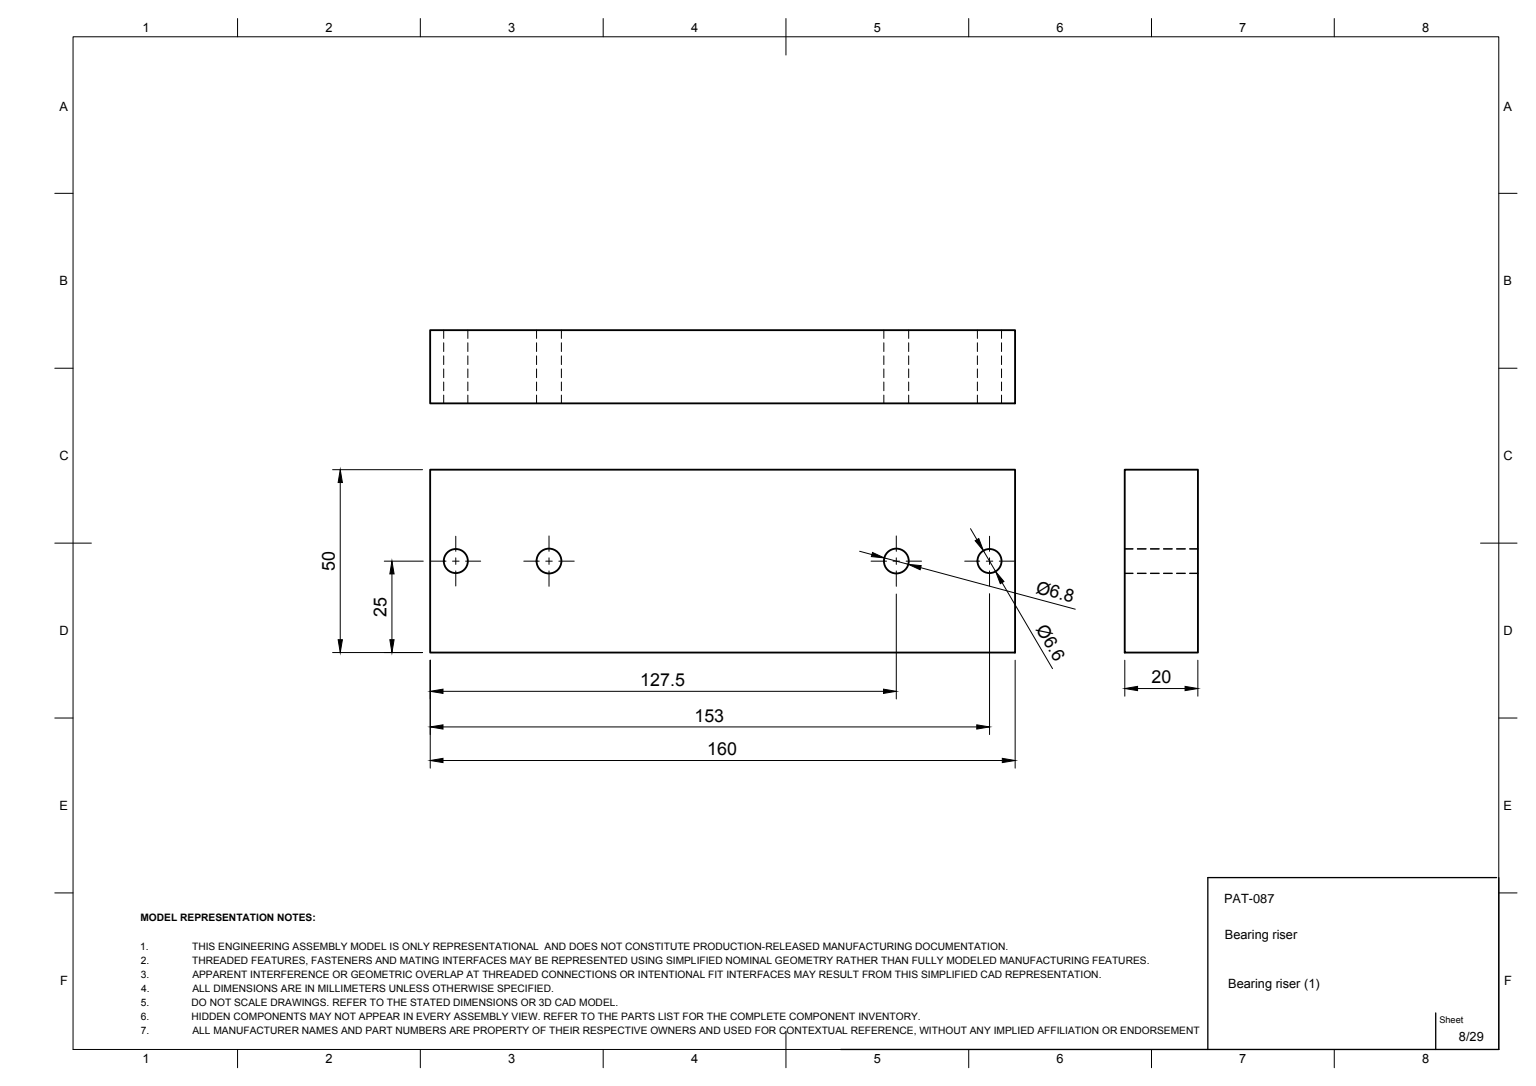
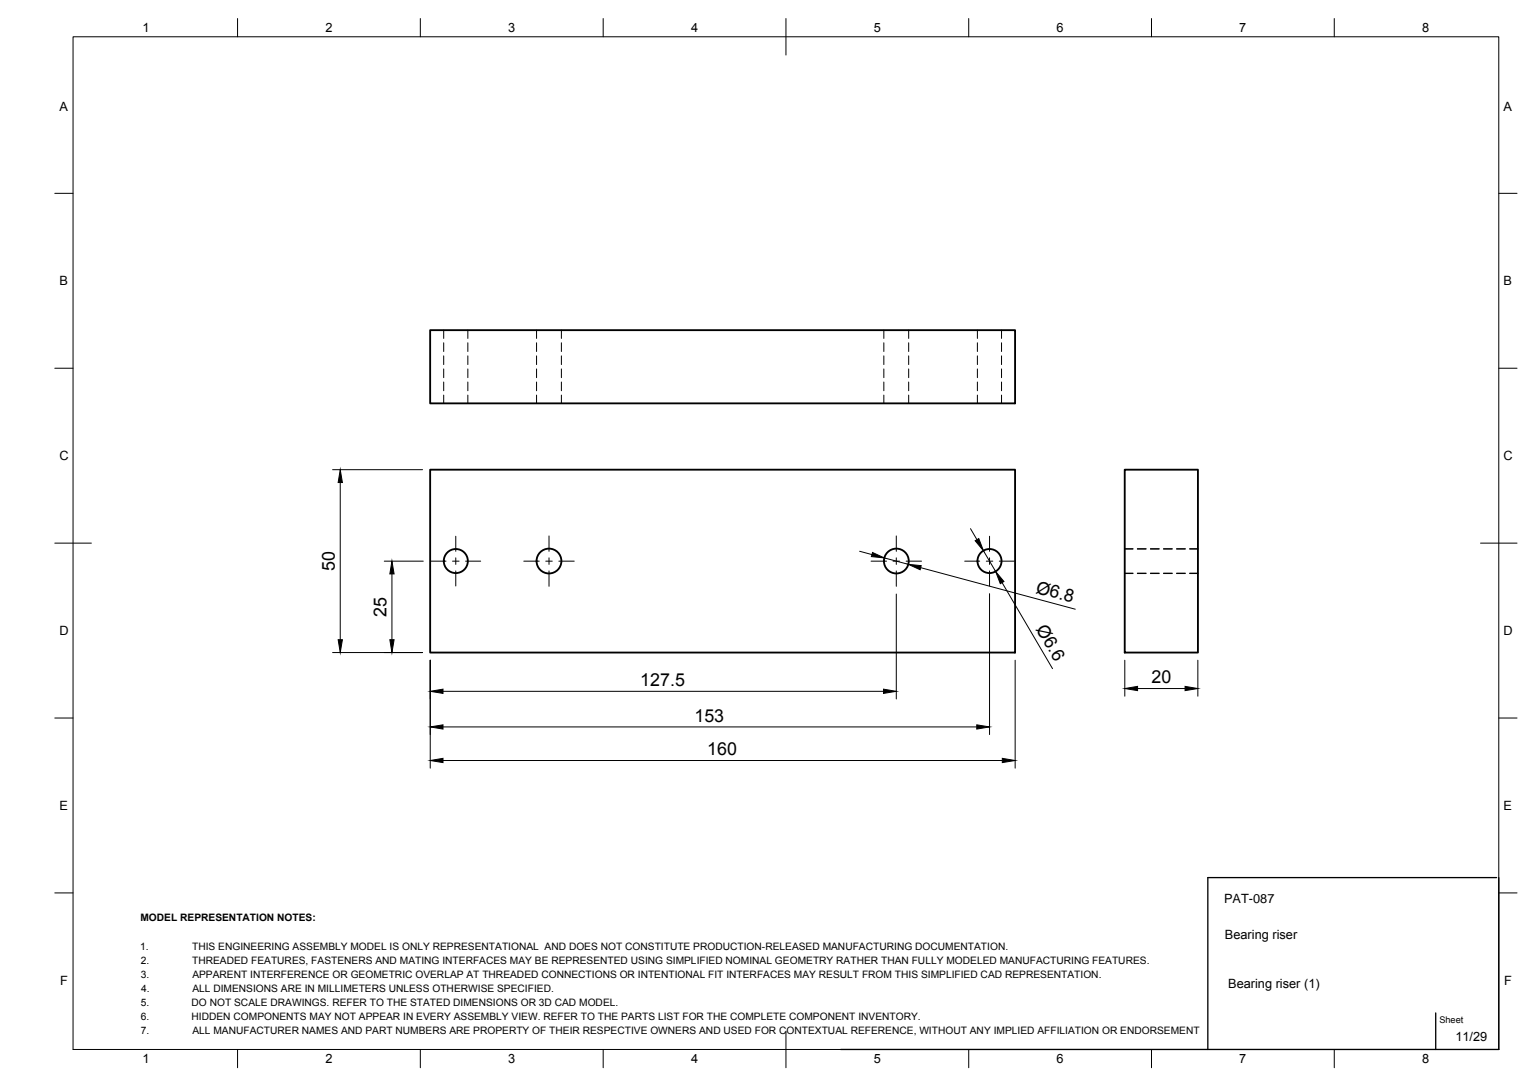
ISO-10303-21;
HEADER;
/* Generated by software containing ST-Developer
 * from STEP Tools, Inc. (www.steptools.com) 
 */

FILE_DESCRIPTION(
/* description */ ('Rigid flange shaft coupling assembly'),
/* implementation_level */ '2;1');

FILE_NAME(
/* name */ 'Bearing riser.step',
/* time_stamp */ '2026-10-27T10:47:16-07:00',
/* author */ (''),
/* organization */ (''),
/* preprocessor_version */ 'ST-DEVELOPER v20.2',
/* originating_system */ 'Autodesk Translation Framework v15.17.0.0',
/* authorisation */ '');

FILE_SCHEMA (('AUTOMOTIVE_DESIGN { 1 0 10303 214 3 1 1 }'));
ENDSEC;

DATA;
#10=MECHANICAL_DESIGN_GEOMETRIC_PRESENTATION_REPRESENTATION('',(#401),#9141);
#345=SHAPE_REPRESENTATION_RELATIONSHIP('SRR','None',#9279,#373);
#373=ADVANCED_BREP_SHAPE_REPRESENTATION('',(#430),#9114);
#401=STYLED_ITEM('',(#9500),#430);
#430=MANIFOLD_SOLID_BREP('Body1',#4755);
#461=FACE_BOUND('',#1055,.T.);
#462=FACE_BOUND('',#1056,.T.);
#463=FACE_BOUND('',#1057,.T.);
#464=FACE_BOUND('',#1058,.T.);
#465=FACE_BOUND('',#1060,.T.);
#466=FACE_BOUND('',#1061,.T.);
#467=FACE_BOUND('',#1062,.T.);
#468=FACE_BOUND('',#1063,.T.);
#588=PLANE('',#5141);
#589=PLANE('',#5142);
#590=PLANE('',#5143);
#591=PLANE('',#5144);
#592=PLANE('',#5145);
#593=PLANE('',#5146);
#766=FACE_OUTER_BOUND('',#1046,.T.);
#767=FACE_OUTER_BOUND('',#1047,.T.);
#768=FACE_OUTER_BOUND('',#1048,.T.);
#769=FACE_OUTER_BOUND('',#1049,.T.);
#770=FACE_OUTER_BOUND('',#1050,.T.);
#771=FACE_OUTER_BOUND('',#1051,.T.);
#772=FACE_OUTER_BOUND('',#1052,.T.);
#773=FACE_OUTER_BOUND('',#1053,.T.);
#774=FACE_OUTER_BOUND('',#1054,.T.);
#775=FACE_OUTER_BOUND('',#1059,.T.);
#1046=EDGE_LOOP('',(#3339,#3340,#3341,#3342));
#1047=EDGE_LOOP('',(#3343,#3344,#3345,#3346));
#1048=EDGE_LOOP('',(#3347,#3348,#3349,#3350));
#1049=EDGE_LOOP('',(#3351,#3352,#3353,#3354));
#1050=EDGE_LOOP('',(#3355,#3356,#3357,#3358));
#1051=EDGE_LOOP('',(#3359,#3360,#3361,#3362));
#1052=EDGE_LOOP('',(#3363,#3364,#3365,#3366));
#1053=EDGE_LOOP('',(#3367,#3368,#3369,#3370));
#1054=EDGE_LOOP('',(#3371,#3372,#3373,#3374));
#1055=EDGE_LOOP('',(#3375));
#1056=EDGE_LOOP('',(#3376));
#1057=EDGE_LOOP('',(#3377));
#1058=EDGE_LOOP('',(#3378));
#1059=EDGE_LOOP('',(#3379,#3380,#3381,#3382));
#1060=EDGE_LOOP('',(#3383));
#1061=EDGE_LOOP('',(#3384));
#1062=EDGE_LOOP('',(#3385));
#1063=EDGE_LOOP('',(#3386));
#1445=LINE('',#7197,#1790);
#1446=LINE('',#7203,#1791);
#1447=LINE('',#7209,#1792);
#1448=LINE('',#7215,#1793);
#1449=LINE('',#7220,#1794);
#1450=LINE('',#7222,#1795);
#1451=LINE('',#7224,#1796);
#1452=LINE('',#7225,#1797);
#1453=LINE('',#7228,#1798);
#1454=LINE('',#7230,#1799);
#1455=LINE('',#7231,#1800);
#1456=LINE('',#7234,#1801);
#1457=LINE('',#7236,#1802);
#1458=LINE('',#7237,#1803);
#1459=LINE('',#7239,#1804);
#1460=LINE('',#7240,#1805);
#1790=VECTOR('',#5758,0.34);
#1791=VECTOR('',#5765,0.34);
#1792=VECTOR('',#5772,0.33);
#1793=VECTOR('',#5779,0.33);
#1794=VECTOR('',#5784,1.);
#1795=VECTOR('',#5785,1.);
#1796=VECTOR('',#5786,1.);
#1797=VECTOR('',#5787,1.);
#1798=VECTOR('',#5790,1.);
#1799=VECTOR('',#5791,1.);
#1800=VECTOR('',#5792,1.);
#1801=VECTOR('',#5795,1.);
#1802=VECTOR('',#5796,1.);
#1803=VECTOR('',#5797,1.);
#1804=VECTOR('',#5800,1.);
#1805=VECTOR('',#5801,1.);
#2103=CIRCLE('',#5130,0.34);
#2104=CIRCLE('',#5131,0.34);
#2105=CIRCLE('',#5133,0.34);
#2106=CIRCLE('',#5134,0.34);
#2107=CIRCLE('',#5136,0.33);
#2108=CIRCLE('',#5137,0.33);
#2109=CIRCLE('',#5139,0.33);
#2110=CIRCLE('',#5140,0.33);
#2308=VERTEX_POINT('',#7194);
#2309=VERTEX_POINT('',#7196);
#2310=VERTEX_POINT('',#7200);
#2311=VERTEX_POINT('',#7202);
#2312=VERTEX_POINT('',#7206);
#2313=VERTEX_POINT('',#7208);
#2314=VERTEX_POINT('',#7212);
#2315=VERTEX_POINT('',#7214);
#2316=VERTEX_POINT('',#7218);
#2317=VERTEX_POINT('',#7219);
#2318=VERTEX_POINT('',#7221);
#2319=VERTEX_POINT('',#7223);
#2320=VERTEX_POINT('',#7227);
#2321=VERTEX_POINT('',#7229);
#2322=VERTEX_POINT('',#7233);
#2323=VERTEX_POINT('',#7235);
#2713=EDGE_CURVE('',#2308,#2308,#2103,.T.);
#2714=EDGE_CURVE('',#2308,#2309,#1445,.T.);
#2715=EDGE_CURVE('',#2309,#2309,#2104,.T.);
#2716=EDGE_CURVE('',#2310,#2310,#2105,.T.);
#2717=EDGE_CURVE('',#2310,#2311,#1446,.T.);
#2718=EDGE_CURVE('',#2311,#2311,#2106,.T.);
#2719=EDGE_CURVE('',#2312,#2312,#2107,.T.);
#2720=EDGE_CURVE('',#2312,#2313,#1447,.T.);
#2721=EDGE_CURVE('',#2313,#2313,#2108,.T.);
#2722=EDGE_CURVE('',#2314,#2314,#2109,.T.);
#2723=EDGE_CURVE('',#2314,#2315,#1448,.T.);
#2724=EDGE_CURVE('',#2315,#2315,#2110,.T.);
#2725=EDGE_CURVE('',#2316,#2317,#1449,.T.);
#2726=EDGE_CURVE('',#2317,#2318,#1450,.T.);
#2727=EDGE_CURVE('',#2319,#2318,#1451,.T.);
#2728=EDGE_CURVE('',#2316,#2319,#1452,.T.);
#2729=EDGE_CURVE('',#2320,#2316,#1453,.T.);
#2730=EDGE_CURVE('',#2321,#2319,#1454,.T.);
#2731=EDGE_CURVE('',#2320,#2321,#1455,.T.);
#2732=EDGE_CURVE('',#2322,#2320,#1456,.T.);
#2733=EDGE_CURVE('',#2323,#2321,#1457,.T.);
#2734=EDGE_CURVE('',#2322,#2323,#1458,.T.);
#2735=EDGE_CURVE('',#2317,#2322,#1459,.T.);
#2736=EDGE_CURVE('',#2318,#2323,#1460,.T.);
#3339=ORIENTED_EDGE('',*,*,#2713,.F.);
#3340=ORIENTED_EDGE('',*,*,#2714,.T.);
#3341=ORIENTED_EDGE('',*,*,#2715,.F.);
#3342=ORIENTED_EDGE('',*,*,#2714,.F.);
#3343=ORIENTED_EDGE('',*,*,#2716,.F.);
#3344=ORIENTED_EDGE('',*,*,#2717,.T.);
#3345=ORIENTED_EDGE('',*,*,#2718,.F.);
#3346=ORIENTED_EDGE('',*,*,#2717,.F.);
#3347=ORIENTED_EDGE('',*,*,#2719,.F.);
#3348=ORIENTED_EDGE('',*,*,#2720,.T.);
#3349=ORIENTED_EDGE('',*,*,#2721,.F.);
#3350=ORIENTED_EDGE('',*,*,#2720,.F.);
#3351=ORIENTED_EDGE('',*,*,#2722,.F.);
#3352=ORIENTED_EDGE('',*,*,#2723,.T.);
#3353=ORIENTED_EDGE('',*,*,#2724,.F.);
#3354=ORIENTED_EDGE('',*,*,#2723,.F.);
#3355=ORIENTED_EDGE('',*,*,#2725,.T.);
#3356=ORIENTED_EDGE('',*,*,#2726,.T.);
#3357=ORIENTED_EDGE('',*,*,#2727,.F.);
#3358=ORIENTED_EDGE('',*,*,#2728,.F.);
#3359=ORIENTED_EDGE('',*,*,#2729,.T.);
#3360=ORIENTED_EDGE('',*,*,#2728,.T.);
#3361=ORIENTED_EDGE('',*,*,#2730,.F.);
#3362=ORIENTED_EDGE('',*,*,#2731,.F.);
#3363=ORIENTED_EDGE('',*,*,#2732,.T.);
#3364=ORIENTED_EDGE('',*,*,#2731,.T.);
#3365=ORIENTED_EDGE('',*,*,#2733,.F.);
#3366=ORIENTED_EDGE('',*,*,#2734,.F.);
#3367=ORIENTED_EDGE('',*,*,#2735,.T.);
#3368=ORIENTED_EDGE('',*,*,#2734,.T.);
#3369=ORIENTED_EDGE('',*,*,#2736,.F.);
#3370=ORIENTED_EDGE('',*,*,#2726,.F.);
#3371=ORIENTED_EDGE('',*,*,#2736,.T.);
#3372=ORIENTED_EDGE('',*,*,#2733,.T.);
#3373=ORIENTED_EDGE('',*,*,#2730,.T.);
#3374=ORIENTED_EDGE('',*,*,#2727,.T.);
#3375=ORIENTED_EDGE('',*,*,#2715,.T.);
#3376=ORIENTED_EDGE('',*,*,#2718,.T.);
#3377=ORIENTED_EDGE('',*,*,#2721,.T.);
#3378=ORIENTED_EDGE('',*,*,#2724,.T.);
#3379=ORIENTED_EDGE('',*,*,#2735,.F.);
#3380=ORIENTED_EDGE('',*,*,#2725,.F.);
#3381=ORIENTED_EDGE('',*,*,#2729,.F.);
#3382=ORIENTED_EDGE('',*,*,#2732,.F.);
#3383=ORIENTED_EDGE('',*,*,#2713,.T.);
#3384=ORIENTED_EDGE('',*,*,#2716,.T.);
#3385=ORIENTED_EDGE('',*,*,#2719,.T.);
#3386=ORIENTED_EDGE('',*,*,#2722,.T.);
#4403=CYLINDRICAL_SURFACE('',#5129,0.34);
#4404=CYLINDRICAL_SURFACE('',#5132,0.34);
#4405=CYLINDRICAL_SURFACE('',#5135,0.33);
#4406=CYLINDRICAL_SURFACE('',#5138,0.33);
#4502=ADVANCED_FACE('',(#766),#4403,.F.);
#4503=ADVANCED_FACE('',(#767),#4404,.F.);
#4504=ADVANCED_FACE('',(#768),#4405,.F.);
#4505=ADVANCED_FACE('',(#769),#4406,.F.);
#4506=ADVANCED_FACE('',(#770),#588,.T.);
#4507=ADVANCED_FACE('',(#771),#589,.T.);
#4508=ADVANCED_FACE('',(#772),#590,.T.);
#4509=ADVANCED_FACE('',(#773),#591,.T.);
#4510=ADVANCED_FACE('',(#774,#461,#462,#463,#464),#592,.T.);
#4511=ADVANCED_FACE('',(#775,#465,#466,#467,#468),#593,.F.);
#4755=CLOSED_SHELL('',(#4502,#4503,#4504,#4505,#4506,#4507,#4508,#4509,
#4510,#4511));
#5128=AXIS2_PLACEMENT_3D('',#7192,#5752,#5753);
#5129=AXIS2_PLACEMENT_3D('',#7193,#5754,#5755);
#5130=AXIS2_PLACEMENT_3D('',#7195,#5756,#5757);
#5131=AXIS2_PLACEMENT_3D('',#7198,#5759,#5760);
#5132=AXIS2_PLACEMENT_3D('',#7199,#5761,#5762);
#5133=AXIS2_PLACEMENT_3D('',#7201,#5763,#5764);
#5134=AXIS2_PLACEMENT_3D('',#7204,#5766,#5767);
#5135=AXIS2_PLACEMENT_3D('',#7205,#5768,#5769);
#5136=AXIS2_PLACEMENT_3D('',#7207,#5770,#5771);
#5137=AXIS2_PLACEMENT_3D('',#7210,#5773,#5774);
#5138=AXIS2_PLACEMENT_3D('',#7211,#5775,#5776);
#5139=AXIS2_PLACEMENT_3D('',#7213,#5777,#5778);
#5140=AXIS2_PLACEMENT_3D('',#7216,#5780,#5781);
#5141=AXIS2_PLACEMENT_3D('',#7217,#5782,#5783);
#5142=AXIS2_PLACEMENT_3D('',#7226,#5788,#5789);
#5143=AXIS2_PLACEMENT_3D('',#7232,#5793,#5794);
#5144=AXIS2_PLACEMENT_3D('',#7238,#5798,#5799);
#5145=AXIS2_PLACEMENT_3D('',#7241,#5802,#5803);
#5146=AXIS2_PLACEMENT_3D('',#7242,#5804,#5805);
#5752=DIRECTION('axis',(0.,0.,1.));
#5753=DIRECTION('refdir',(1.,0.,0.));
#5754=DIRECTION('center_axis',(0.,0.,1.));
#5755=DIRECTION('ref_axis',(1.,0.,0.));
#5756=DIRECTION('center_axis',(0.,0.,1.));
#5757=DIRECTION('ref_axis',(1.,0.,0.));
#5758=DIRECTION('',(0.,0.,1.));
#5759=DIRECTION('center_axis',(0.,0.,-1.));
#5760=DIRECTION('ref_axis',(1.,0.,0.));
#5761=DIRECTION('center_axis',(0.,0.,1.));
#5762=DIRECTION('ref_axis',(1.,0.,0.));
#5763=DIRECTION('center_axis',(0.,0.,1.));
#5764=DIRECTION('ref_axis',(1.,0.,0.));
#5765=DIRECTION('',(0.,0.,1.));
#5766=DIRECTION('center_axis',(0.,0.,-1.));
#5767=DIRECTION('ref_axis',(1.,0.,0.));
#5768=DIRECTION('center_axis',(0.,0.,1.));
#5769=DIRECTION('ref_axis',(1.,0.,0.));
#5770=DIRECTION('center_axis',(0.,0.,1.));
#5771=DIRECTION('ref_axis',(1.,0.,0.));
#5772=DIRECTION('',(0.,0.,1.));
#5773=DIRECTION('center_axis',(0.,0.,-1.));
#5774=DIRECTION('ref_axis',(1.,0.,0.));
#5775=DIRECTION('center_axis',(0.,0.,1.));
#5776=DIRECTION('ref_axis',(1.,0.,0.));
#5777=DIRECTION('center_axis',(0.,0.,1.));
#5778=DIRECTION('ref_axis',(1.,0.,0.));
#5779=DIRECTION('',(0.,0.,1.));
#5780=DIRECTION('center_axis',(0.,0.,-1.));
#5781=DIRECTION('ref_axis',(1.,0.,0.));
#5782=DIRECTION('center_axis',(0.,1.,0.));
#5783=DIRECTION('ref_axis',(-1.,0.,0.));
#5784=DIRECTION('',(-1.,0.,0.));
#5785=DIRECTION('',(0.,0.,1.));
#5786=DIRECTION('',(-1.,0.,0.));
#5787=DIRECTION('',(0.,0.,1.));
#5788=DIRECTION('center_axis',(1.,0.,0.));
#5789=DIRECTION('ref_axis',(0.,1.,0.));
#5790=DIRECTION('',(0.,1.,0.));
#5791=DIRECTION('',(0.,1.,0.));
#5792=DIRECTION('',(0.,0.,1.));
#5793=DIRECTION('center_axis',(0.,-1.,0.));
#5794=DIRECTION('ref_axis',(1.,0.,0.));
#5795=DIRECTION('',(1.,0.,0.));
#5796=DIRECTION('',(1.,0.,0.));
#5797=DIRECTION('',(0.,0.,1.));
#5798=DIRECTION('center_axis',(-1.,0.,0.));
#5799=DIRECTION('ref_axis',(0.,-1.,0.));
#5800=DIRECTION('',(0.,-1.,0.));
#5801=DIRECTION('',(0.,-1.,0.));
#5802=DIRECTION('center_axis',(0.,0.,1.));
#5803=DIRECTION('ref_axis',(1.,0.,0.));
#5804=DIRECTION('center_axis',(0.,0.,1.));
#5805=DIRECTION('ref_axis',(1.,0.,0.));
#7192=CARTESIAN_POINT('',(0.,0.,0.));
#7193=CARTESIAN_POINT('Origin',(-4.75,0.,1.1));
#7194=CARTESIAN_POINT('',(-5.09,-4.163799117101E-17,1.2));
#7195=CARTESIAN_POINT('Origin',(-4.75,0.,1.2));
#7196=CARTESIAN_POINT('',(-5.09,4.163799117101E-17,3.2));
#7197=CARTESIAN_POINT('',(-5.09,-4.163799117101E-17,1.1));
#7198=CARTESIAN_POINT('Origin',(-4.75,0.,3.2));
#7199=CARTESIAN_POINT('Origin',(4.75,0.,1.1));
#7200=CARTESIAN_POINT('',(4.41,-4.163799117101E-17,1.2));
#7201=CARTESIAN_POINT('Origin',(4.75,0.,1.2));
#7202=CARTESIAN_POINT('',(4.41,4.163799117101E-17,3.2));
#7203=CARTESIAN_POINT('',(4.41,-4.163799117101E-17,1.1));
#7204=CARTESIAN_POINT('Origin',(4.75,0.,3.2));
#7205=CARTESIAN_POINT('Origin',(-7.3,0.,1.1));
#7206=CARTESIAN_POINT('',(-7.63,-4.04133443718627E-17,1.2));
#7207=CARTESIAN_POINT('Origin',(-7.3,0.,1.2));
#7208=CARTESIAN_POINT('',(-7.63,4.04133443718627E-17,3.2));
#7209=CARTESIAN_POINT('',(-7.63,-4.04133443718627E-17,1.1));
#7210=CARTESIAN_POINT('Origin',(-7.3,0.,3.2));
#7211=CARTESIAN_POINT('Origin',(7.3,0.,1.1));
#7212=CARTESIAN_POINT('',(6.97,-4.04133443718627E-17,1.2));
#7213=CARTESIAN_POINT('Origin',(7.3,0.,1.2));
#7214=CARTESIAN_POINT('',(6.97,4.04133443718627E-17,3.2));
#7215=CARTESIAN_POINT('',(6.97,-4.04133443718627E-17,1.1));
#7216=CARTESIAN_POINT('Origin',(7.3,0.,3.2));
#7217=CARTESIAN_POINT('Origin',(8.,2.5,1.2));
#7218=CARTESIAN_POINT('',(8.,2.5,1.2));
#7219=CARTESIAN_POINT('',(-8.,2.5,1.2));
#7220=CARTESIAN_POINT('',(8.,2.5,1.2));
#7221=CARTESIAN_POINT('',(-8.,2.5,3.2));
#7222=CARTESIAN_POINT('',(-8.,2.5,1.2));
#7223=CARTESIAN_POINT('',(8.,2.5,3.2));
#7224=CARTESIAN_POINT('',(8.,2.5,3.2));
#7225=CARTESIAN_POINT('',(8.,2.5,1.2));
#7226=CARTESIAN_POINT('Origin',(8.,-2.5,1.2));
#7227=CARTESIAN_POINT('',(8.,-2.5,1.2));
#7228=CARTESIAN_POINT('',(8.,-2.5,1.2));
#7229=CARTESIAN_POINT('',(8.,-2.5,3.2));
#7230=CARTESIAN_POINT('',(8.,-2.5,3.2));
#7231=CARTESIAN_POINT('',(8.,-2.5,1.2));
#7232=CARTESIAN_POINT('Origin',(-8.,-2.5,1.2));
#7233=CARTESIAN_POINT('',(-8.,-2.5,1.2));
#7234=CARTESIAN_POINT('',(-8.,-2.5,1.2));
#7235=CARTESIAN_POINT('',(-8.,-2.5,3.2));
#7236=CARTESIAN_POINT('',(-8.,-2.5,3.2));
#7237=CARTESIAN_POINT('',(-8.,-2.5,1.2));
#7238=CARTESIAN_POINT('Origin',(-8.,2.5,1.2));
#7239=CARTESIAN_POINT('',(-8.,2.5,1.2));
#7240=CARTESIAN_POINT('',(-8.,2.5,3.2));
#7241=CARTESIAN_POINT('Origin',(0.,0.,3.2));
#7242=CARTESIAN_POINT('Origin',(0.,0.,1.2));
#9081=UNCERTAINTY_MEASURE_WITH_UNIT(LENGTH_MEASURE(0.001),#9142,
'DISTANCE_ACCURACY_VALUE',
'Maximum model space distance between geometric entities at asserted c
onnectivities');
#9108=UNCERTAINTY_MEASURE_WITH_UNIT(LENGTH_MEASURE(0.001),#9142,
'DISTANCE_ACCURACY_VALUE',
'Maximum model space distance between geometric entities at asserted c
onnectivities');
#9114=(
GEOMETRIC_REPRESENTATION_CONTEXT(3)
GLOBAL_UNCERTAINTY_ASSIGNED_CONTEXT((#9081))
GLOBAL_UNIT_ASSIGNED_CONTEXT((#9142,#9144,#9145))
REPRESENTATION_CONTEXT('','3D')
);
#9141=(
GEOMETRIC_REPRESENTATION_CONTEXT(3)
GLOBAL_UNCERTAINTY_ASSIGNED_CONTEXT((#9108))
GLOBAL_UNIT_ASSIGNED_CONTEXT((#9142,#9144,#9145))
REPRESENTATION_CONTEXT('','3D')
);
#9142=(
LENGTH_UNIT()
NAMED_UNIT(*)
SI_UNIT(.CENTI.,.METRE.)
);
#9144=(
NAMED_UNIT(*)
PLANE_ANGLE_UNIT()
SI_UNIT($,.RADIAN.)
);
#9145=(
NAMED_UNIT(*)
SI_UNIT($,.STERADIAN.)
SOLID_ANGLE_UNIT()
);
#9151=SHAPE_DEFINITION_REPRESENTATION(#9183,#9279);
#9183=PRODUCT_DEFINITION_SHAPE('',$,#9312);
#9279=SHAPE_REPRESENTATION('',(#5128),#9114);
#9306=PRODUCT_DEFINITION_CONTEXT('part definition',#9404,'design');
#9312=PRODUCT_DEFINITION('Bearing riser','Bearing riser',#9344,#9306);
#9344=PRODUCT_DEFINITION_FORMATION('',$,#9411);
#9404=APPLICATION_CONTEXT(
'Core Data for Automotive Mechanical Design Process');
#9405=PRODUCT_CONTEXT('part definition',#9404,'mechanical');
#9411=PRODUCT('Bearing riser','Bearing riser','Bearing riser',(#9405));
#9494=COLOUR_RGB('Grey',0.48,0.52,0.57);
#9495=FILL_AREA_STYLE_COLOUR('',#9494);
#9496=FILL_AREA_STYLE('',(#9495));
#9497=SURFACE_STYLE_FILL_AREA(#9496);
#9498=SURFACE_SIDE_STYLE('',(#9497));
#9499=SURFACE_STYLE_USAGE(.BOTH.,#9498);
#9500=PRESENTATION_STYLE_ASSIGNMENT((#9499));
ENDSEC;
END-ISO-10303-21;
